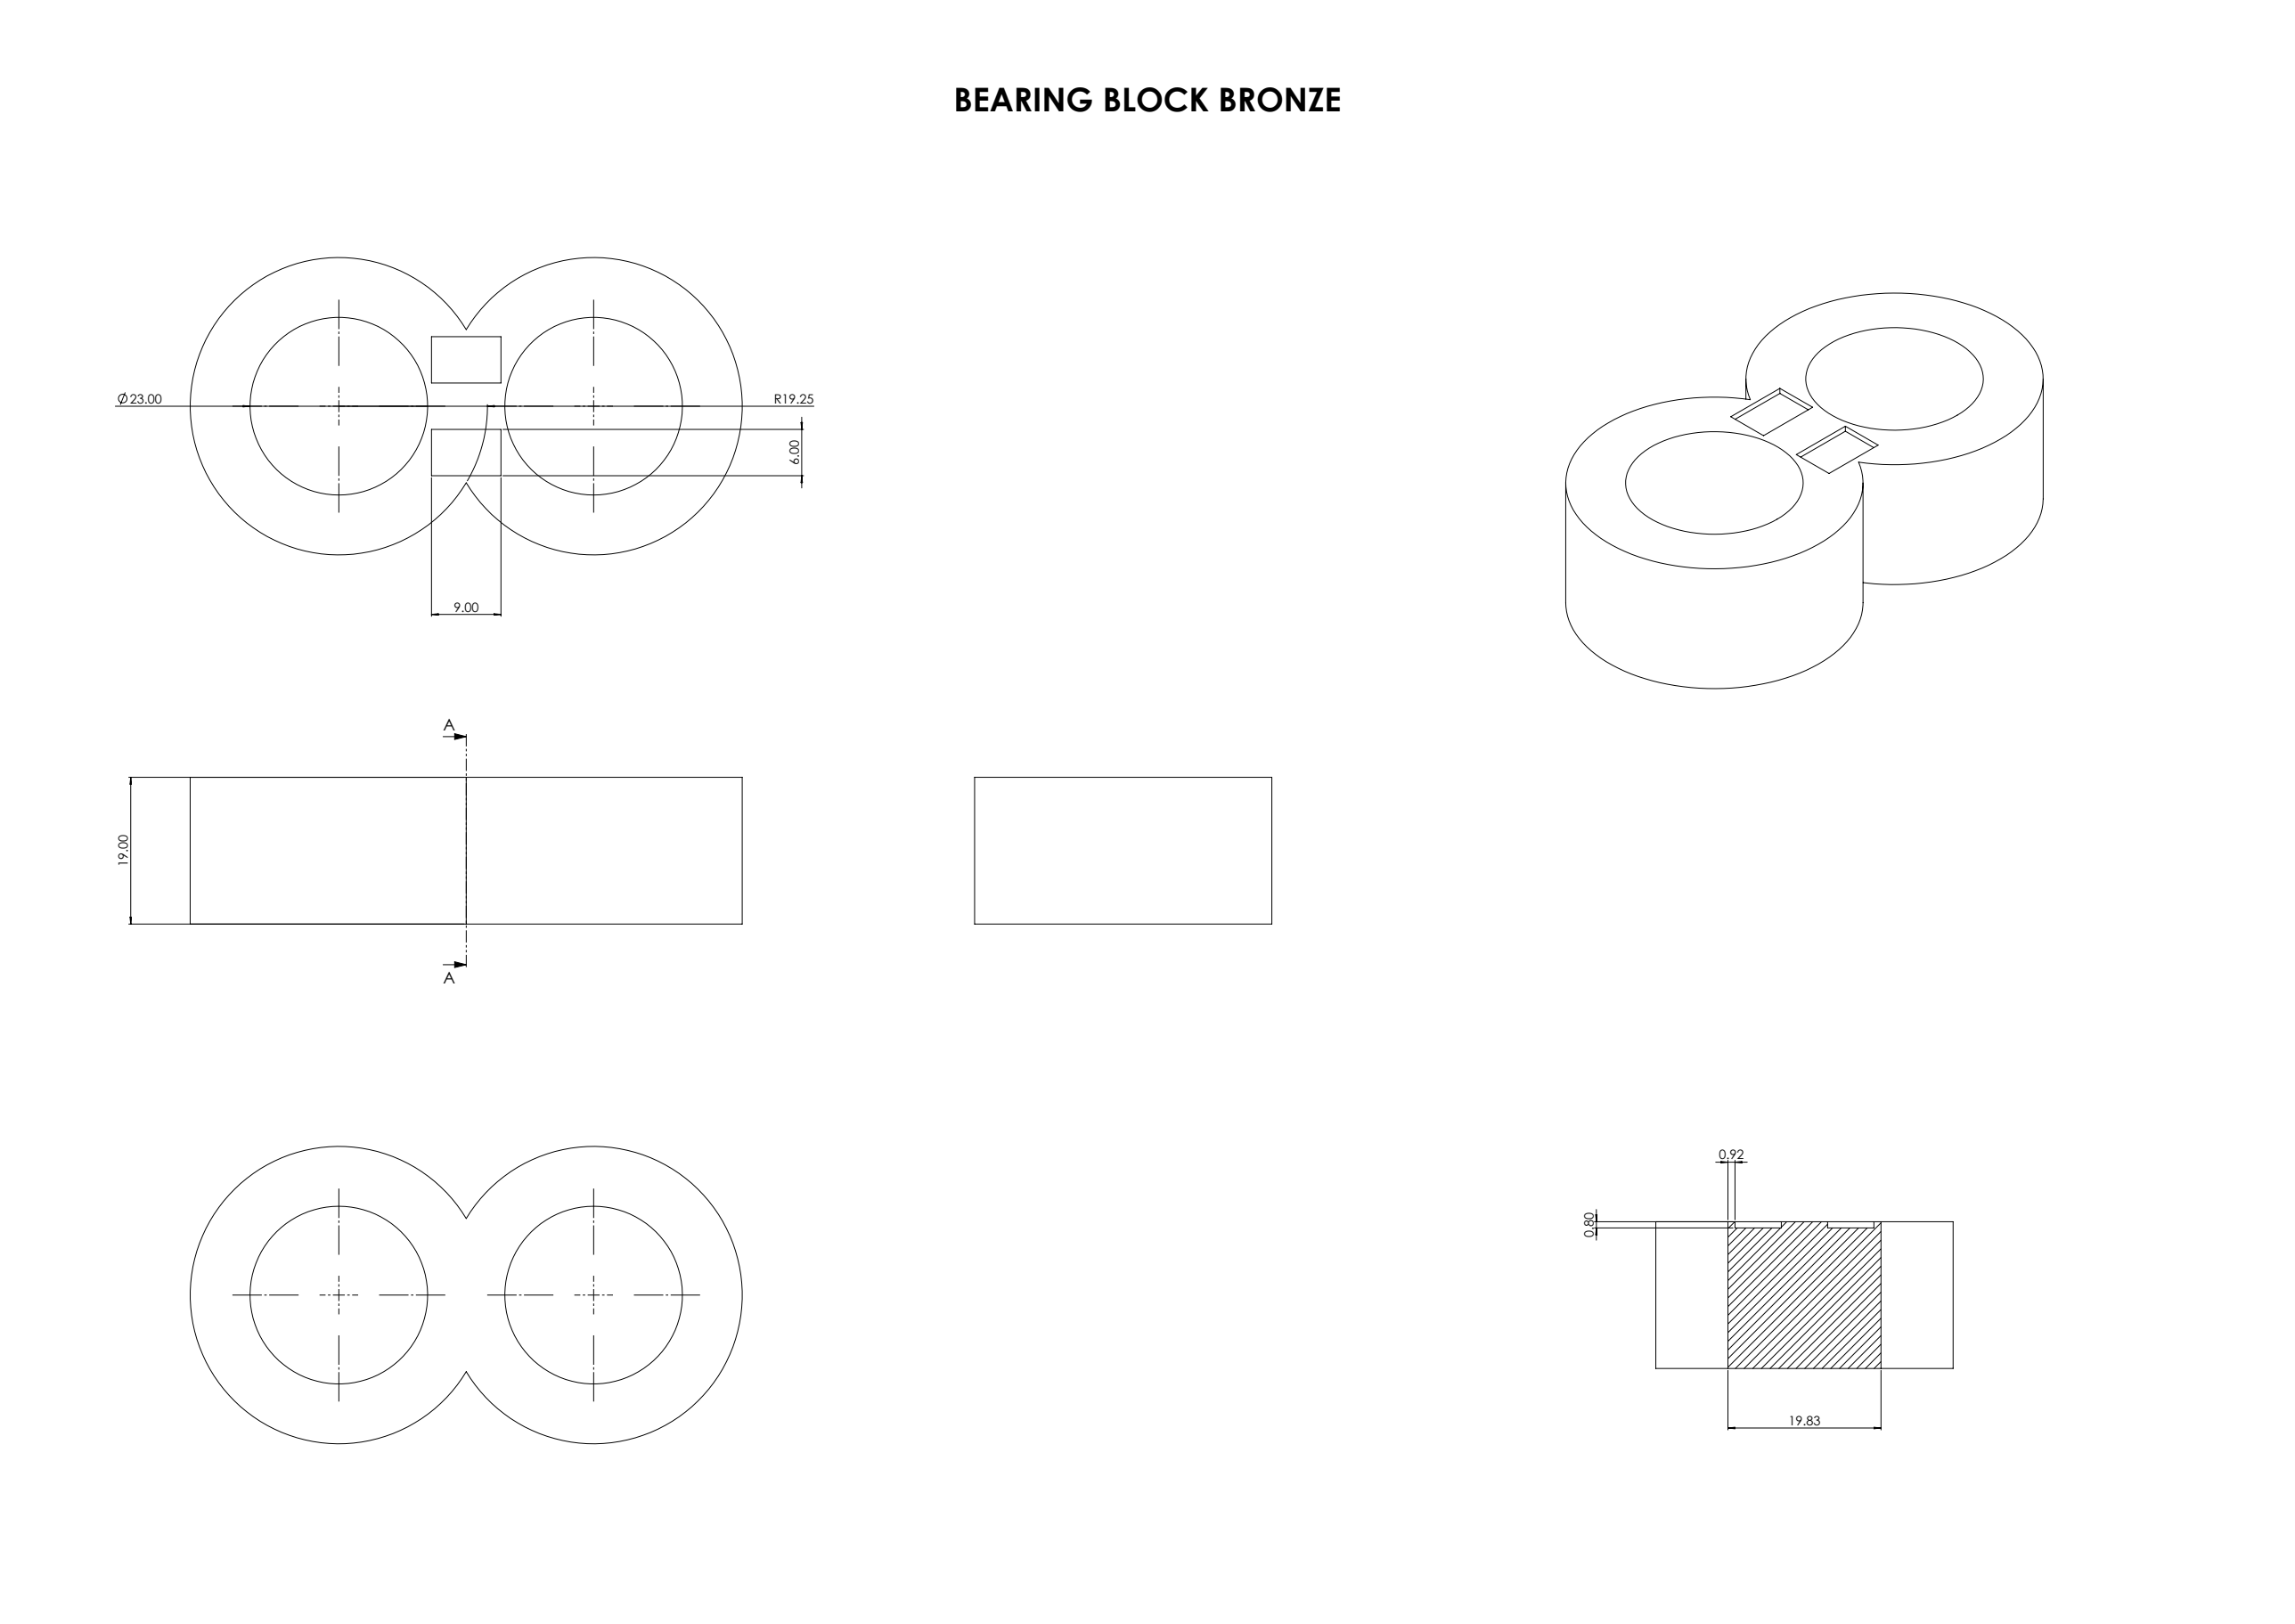
ISO-10303-21;
HEADER;
/* Generated by software containing ST-Developer
 * from STEP Tools, Inc. (www.steptools.com) 
 */

FILE_DESCRIPTION(
/* description */ (''),
/* implementation_level */ '2;1');

FILE_NAME(
/* name */ '06_Bearing_Block_Bronze.step',
/* time_stamp */ '2026-10-26T06:59:52-07:00',
/* author */ (''),
/* organization */ (''),
/* preprocessor_version */ 'ST-DEVELOPER v20.2',
/* originating_system */ 'Autodesk Translation Framework v15.15.0.0',
/* authorisation */ '');

FILE_SCHEMA (('AUTOMOTIVE_DESIGN { 1 0 10303 214 3 1 1 }'));
ENDSEC;

DATA;
#10=MECHANICAL_DESIGN_GEOMETRIC_PRESENTATION_REPRESENTATION('',(#169),#46395);
#141=SHAPE_REPRESENTATION_RELATIONSHIP('SRR','None',#46461,#155);
#155=ADVANCED_BREP_SHAPE_REPRESENTATION('',(#183),#46386);
#169=STYLED_ITEM('',(#46596),#183);
#183=MANIFOLD_SOLID_BREP('Body1',#24942);
#519=CYLINDRICAL_SURFACE('',#26421,11.5);
#520=CYLINDRICAL_SURFACE('',#26424,11.5);
#521=CYLINDRICAL_SURFACE('',#26427,19.25);
#522=CYLINDRICAL_SURFACE('',#26430,19.25);
#651=FACE_BOUND('',#4155,.T.);
#652=FACE_BOUND('',#4156,.T.);
#653=FACE_BOUND('',#4157,.T.);
#654=FACE_BOUND('',#4158,.T.);
#655=FACE_BOUND('',#4160,.T.);
#656=FACE_BOUND('',#4161,.T.);
#1500=PLANE('',#26411);
#1501=PLANE('',#26412);
#1502=PLANE('',#26413);
#1503=PLANE('',#26414);
#1504=PLANE('',#26415);
#1505=PLANE('',#26416);
#1506=PLANE('',#26417);
#1507=PLANE('',#26418);
#1508=PLANE('',#26419);
#1509=PLANE('',#26420);
#1510=PLANE('',#26433);
#1511=PLANE('',#26434);
#2744=FACE_OUTER_BOUND('',#4140,.T.);
#2745=FACE_OUTER_BOUND('',#4141,.T.);
#2746=FACE_OUTER_BOUND('',#4142,.T.);
#2747=FACE_OUTER_BOUND('',#4143,.T.);
#2748=FACE_OUTER_BOUND('',#4144,.T.);
#2749=FACE_OUTER_BOUND('',#4145,.T.);
#2750=FACE_OUTER_BOUND('',#4146,.T.);
#2751=FACE_OUTER_BOUND('',#4147,.T.);
#2752=FACE_OUTER_BOUND('',#4148,.T.);
#2753=FACE_OUTER_BOUND('',#4149,.T.);
#2754=FACE_OUTER_BOUND('',#4150,.T.);
#2755=FACE_OUTER_BOUND('',#4151,.T.);
#2756=FACE_OUTER_BOUND('',#4152,.T.);
#2757=FACE_OUTER_BOUND('',#4153,.T.);
#2758=FACE_OUTER_BOUND('',#4154,.T.);
#2759=FACE_OUTER_BOUND('',#4159,.T.);
#4140=EDGE_LOOP('',(#22016,#22017,#22018,#22019));
#4141=EDGE_LOOP('',(#22020,#22021,#22022,#22023));
#4142=EDGE_LOOP('',(#22024,#22025,#22026,#22027));
#4143=EDGE_LOOP('',(#22028,#22029,#22030,#22031));
#4144=EDGE_LOOP('',(#22032,#22033,#22034,#22035));
#4145=EDGE_LOOP('',(#22036,#22037,#22038,#22039));
#4146=EDGE_LOOP('',(#22040,#22041,#22042,#22043));
#4147=EDGE_LOOP('',(#22044,#22045,#22046,#22047));
#4148=EDGE_LOOP('',(#22048,#22049,#22050,#22051));
#4149=EDGE_LOOP('',(#22052,#22053,#22054,#22055));
#4150=EDGE_LOOP('',(#22056,#22057,#22058,#22059));
#4151=EDGE_LOOP('',(#22060,#22061,#22062,#22063));
#4152=EDGE_LOOP('',(#22064,#22065,#22066,#22067));
#4153=EDGE_LOOP('',(#22068,#22069,#22070,#22071));
#4154=EDGE_LOOP('',(#22072,#22073));
#4155=EDGE_LOOP('',(#22074,#22075,#22076,#22077));
#4156=EDGE_LOOP('',(#22078,#22079,#22080,#22081));
#4157=EDGE_LOOP('',(#22082));
#4158=EDGE_LOOP('',(#22083));
#4159=EDGE_LOOP('',(#22084,#22085));
#4160=EDGE_LOOP('',(#22086));
#4161=EDGE_LOOP('',(#22087));
#6899=LINE('',#40133,#9768);
#6900=LINE('',#40135,#9769);
#6901=LINE('',#40137,#9770);
#6902=LINE('',#40138,#9771);
#6903=LINE('',#40141,#9772);
#6904=LINE('',#40143,#9773);
#6905=LINE('',#40144,#9774);
#6906=LINE('',#40147,#9775);
#6907=LINE('',#40149,#9776);
#6908=LINE('',#40150,#9777);
#6909=LINE('',#40152,#9778);
#6910=LINE('',#40153,#9779);
#6911=LINE('',#40158,#9780);
#6912=LINE('',#40160,#9781);
#6913=LINE('',#40162,#9782);
#6914=LINE('',#40163,#9783);
#6915=LINE('',#40166,#9784);
#6916=LINE('',#40168,#9785);
#6917=LINE('',#40169,#9786);
#6918=LINE('',#40172,#9787);
#6919=LINE('',#40174,#9788);
#6920=LINE('',#40175,#9789);
#6921=LINE('',#40177,#9790);
#6922=LINE('',#40178,#9791);
#6923=LINE('',#40184,#9792);
#6924=LINE('',#40190,#9793);
#6925=LINE('',#40197,#9794);
#6926=LINE('',#40200,#9795);
#9768=VECTOR('',#31910,10.);
#9769=VECTOR('',#31911,10.);
#9770=VECTOR('',#31912,10.);
#9771=VECTOR('',#31913,10.);
#9772=VECTOR('',#31916,10.);
#9773=VECTOR('',#31917,10.);
#9774=VECTOR('',#31918,10.);
#9775=VECTOR('',#31921,10.);
#9776=VECTOR('',#31922,10.);
#9777=VECTOR('',#31923,10.);
#9778=VECTOR('',#31926,10.);
#9779=VECTOR('',#31927,10.);
#9780=VECTOR('',#31932,10.);
#9781=VECTOR('',#31933,10.);
#9782=VECTOR('',#31934,10.);
#9783=VECTOR('',#31935,10.);
#9784=VECTOR('',#31938,10.);
#9785=VECTOR('',#31939,10.);
#9786=VECTOR('',#31940,10.);
#9787=VECTOR('',#31943,10.);
#9788=VECTOR('',#31944,10.);
#9789=VECTOR('',#31945,10.);
#9790=VECTOR('',#31948,10.);
#9791=VECTOR('',#31949,10.);
#9792=VECTOR('',#31956,11.5);
#9793=VECTOR('',#31963,11.5);
#9794=VECTOR('',#31970,10.);
#9795=VECTOR('',#31973,10.);
#10581=CIRCLE('',#26422,11.5);
#10582=CIRCLE('',#26423,11.5);
#10583=CIRCLE('',#26425,11.5);
#10584=CIRCLE('',#26426,11.5);
#10585=CIRCLE('',#26428,19.25);
#10586=CIRCLE('',#26429,19.25);
#10587=CIRCLE('',#26431,19.25);
#10588=CIRCLE('',#26432,19.25);
#12520=VERTEX_POINT('',#40131);
#12521=VERTEX_POINT('',#40132);
#12522=VERTEX_POINT('',#40134);
#12523=VERTEX_POINT('',#40136);
#12524=VERTEX_POINT('',#40140);
#12525=VERTEX_POINT('',#40142);
#12526=VERTEX_POINT('',#40146);
#12527=VERTEX_POINT('',#40148);
#12528=VERTEX_POINT('',#40156);
#12529=VERTEX_POINT('',#40157);
#12530=VERTEX_POINT('',#40159);
#12531=VERTEX_POINT('',#40161);
#12532=VERTEX_POINT('',#40165);
#12533=VERTEX_POINT('',#40167);
#12534=VERTEX_POINT('',#40171);
#12535=VERTEX_POINT('',#40173);
#12536=VERTEX_POINT('',#40181);
#12537=VERTEX_POINT('',#40183);
#12538=VERTEX_POINT('',#40187);
#12539=VERTEX_POINT('',#40189);
#12540=VERTEX_POINT('',#40193);
#12541=VERTEX_POINT('',#40194);
#12542=VERTEX_POINT('',#40196);
#12543=VERTEX_POINT('',#40198);
#15761=EDGE_CURVE('',#12520,#12521,#6899,.T.);
#15762=EDGE_CURVE('',#12520,#12522,#6900,.T.);
#15763=EDGE_CURVE('',#12522,#12523,#6901,.T.);
#15764=EDGE_CURVE('',#12521,#12523,#6902,.T.);
#15765=EDGE_CURVE('',#12524,#12520,#6903,.T.);
#15766=EDGE_CURVE('',#12524,#12525,#6904,.T.);
#15767=EDGE_CURVE('',#12525,#12522,#6905,.T.);
#15768=EDGE_CURVE('',#12526,#12524,#6906,.T.);
#15769=EDGE_CURVE('',#12526,#12527,#6907,.T.);
#15770=EDGE_CURVE('',#12527,#12525,#6908,.T.);
#15771=EDGE_CURVE('',#12521,#12526,#6909,.T.);
#15772=EDGE_CURVE('',#12523,#12527,#6910,.T.);
#15773=EDGE_CURVE('',#12528,#12529,#6911,.T.);
#15774=EDGE_CURVE('',#12528,#12530,#6912,.T.);
#15775=EDGE_CURVE('',#12530,#12531,#6913,.T.);
#15776=EDGE_CURVE('',#12529,#12531,#6914,.T.);
#15777=EDGE_CURVE('',#12532,#12528,#6915,.T.);
#15778=EDGE_CURVE('',#12532,#12533,#6916,.T.);
#15779=EDGE_CURVE('',#12533,#12530,#6917,.T.);
#15780=EDGE_CURVE('',#12534,#12532,#6918,.T.);
#15781=EDGE_CURVE('',#12534,#12535,#6919,.T.);
#15782=EDGE_CURVE('',#12535,#12533,#6920,.T.);
#15783=EDGE_CURVE('',#12529,#12534,#6921,.T.);
#15784=EDGE_CURVE('',#12531,#12535,#6922,.T.);
#15785=EDGE_CURVE('',#12536,#12536,#10581,.T.);
#15786=EDGE_CURVE('',#12536,#12537,#6923,.T.);
#15787=EDGE_CURVE('',#12537,#12537,#10582,.T.);
#15788=EDGE_CURVE('',#12538,#12538,#10583,.T.);
#15789=EDGE_CURVE('',#12538,#12539,#6924,.T.);
#15790=EDGE_CURVE('',#12539,#12539,#10584,.T.);
#15791=EDGE_CURVE('',#12540,#12541,#10585,.T.);
#15792=EDGE_CURVE('',#12541,#12542,#6925,.T.);
#15793=EDGE_CURVE('',#12543,#12542,#10586,.T.);
#15794=EDGE_CURVE('',#12540,#12543,#6926,.T.);
#15795=EDGE_CURVE('',#12541,#12540,#10587,.T.);
#15796=EDGE_CURVE('',#12542,#12543,#10588,.T.);
#22016=ORIENTED_EDGE('',*,*,#15761,.F.);
#22017=ORIENTED_EDGE('',*,*,#15762,.T.);
#22018=ORIENTED_EDGE('',*,*,#15763,.T.);
#22019=ORIENTED_EDGE('',*,*,#15764,.F.);
#22020=ORIENTED_EDGE('',*,*,#15765,.F.);
#22021=ORIENTED_EDGE('',*,*,#15766,.T.);
#22022=ORIENTED_EDGE('',*,*,#15767,.T.);
#22023=ORIENTED_EDGE('',*,*,#15762,.F.);
#22024=ORIENTED_EDGE('',*,*,#15768,.F.);
#22025=ORIENTED_EDGE('',*,*,#15769,.T.);
#22026=ORIENTED_EDGE('',*,*,#15770,.T.);
#22027=ORIENTED_EDGE('',*,*,#15766,.F.);
#22028=ORIENTED_EDGE('',*,*,#15771,.F.);
#22029=ORIENTED_EDGE('',*,*,#15764,.T.);
#22030=ORIENTED_EDGE('',*,*,#15772,.T.);
#22031=ORIENTED_EDGE('',*,*,#15769,.F.);
#22032=ORIENTED_EDGE('',*,*,#15772,.F.);
#22033=ORIENTED_EDGE('',*,*,#15763,.F.);
#22034=ORIENTED_EDGE('',*,*,#15767,.F.);
#22035=ORIENTED_EDGE('',*,*,#15770,.F.);
#22036=ORIENTED_EDGE('',*,*,#15773,.F.);
#22037=ORIENTED_EDGE('',*,*,#15774,.T.);
#22038=ORIENTED_EDGE('',*,*,#15775,.T.);
#22039=ORIENTED_EDGE('',*,*,#15776,.F.);
#22040=ORIENTED_EDGE('',*,*,#15777,.F.);
#22041=ORIENTED_EDGE('',*,*,#15778,.T.);
#22042=ORIENTED_EDGE('',*,*,#15779,.T.);
#22043=ORIENTED_EDGE('',*,*,#15774,.F.);
#22044=ORIENTED_EDGE('',*,*,#15780,.F.);
#22045=ORIENTED_EDGE('',*,*,#15781,.T.);
#22046=ORIENTED_EDGE('',*,*,#15782,.T.);
#22047=ORIENTED_EDGE('',*,*,#15778,.F.);
#22048=ORIENTED_EDGE('',*,*,#15783,.F.);
#22049=ORIENTED_EDGE('',*,*,#15776,.T.);
#22050=ORIENTED_EDGE('',*,*,#15784,.T.);
#22051=ORIENTED_EDGE('',*,*,#15781,.F.);
#22052=ORIENTED_EDGE('',*,*,#15784,.F.);
#22053=ORIENTED_EDGE('',*,*,#15775,.F.);
#22054=ORIENTED_EDGE('',*,*,#15779,.F.);
#22055=ORIENTED_EDGE('',*,*,#15782,.F.);
#22056=ORIENTED_EDGE('',*,*,#15785,.F.);
#22057=ORIENTED_EDGE('',*,*,#15786,.T.);
#22058=ORIENTED_EDGE('',*,*,#15787,.F.);
#22059=ORIENTED_EDGE('',*,*,#15786,.F.);
#22060=ORIENTED_EDGE('',*,*,#15788,.F.);
#22061=ORIENTED_EDGE('',*,*,#15789,.T.);
#22062=ORIENTED_EDGE('',*,*,#15790,.F.);
#22063=ORIENTED_EDGE('',*,*,#15789,.F.);
#22064=ORIENTED_EDGE('',*,*,#15791,.T.);
#22065=ORIENTED_EDGE('',*,*,#15792,.T.);
#22066=ORIENTED_EDGE('',*,*,#15793,.F.);
#22067=ORIENTED_EDGE('',*,*,#15794,.F.);
#22068=ORIENTED_EDGE('',*,*,#15795,.T.);
#22069=ORIENTED_EDGE('',*,*,#15794,.T.);
#22070=ORIENTED_EDGE('',*,*,#15796,.F.);
#22071=ORIENTED_EDGE('',*,*,#15792,.F.);
#22072=ORIENTED_EDGE('',*,*,#15796,.T.);
#22073=ORIENTED_EDGE('',*,*,#15793,.T.);
#22074=ORIENTED_EDGE('',*,*,#15761,.T.);
#22075=ORIENTED_EDGE('',*,*,#15771,.T.);
#22076=ORIENTED_EDGE('',*,*,#15768,.T.);
#22077=ORIENTED_EDGE('',*,*,#15765,.T.);
#22078=ORIENTED_EDGE('',*,*,#15773,.T.);
#22079=ORIENTED_EDGE('',*,*,#15783,.T.);
#22080=ORIENTED_EDGE('',*,*,#15780,.T.);
#22081=ORIENTED_EDGE('',*,*,#15777,.T.);
#22082=ORIENTED_EDGE('',*,*,#15787,.T.);
#22083=ORIENTED_EDGE('',*,*,#15790,.T.);
#22084=ORIENTED_EDGE('',*,*,#15795,.F.);
#22085=ORIENTED_EDGE('',*,*,#15791,.F.);
#22086=ORIENTED_EDGE('',*,*,#15785,.T.);
#22087=ORIENTED_EDGE('',*,*,#15788,.T.);
#24603=ADVANCED_FACE('',(#2744),#1500,.F.);
#24604=ADVANCED_FACE('',(#2745),#1501,.F.);
#24605=ADVANCED_FACE('',(#2746),#1502,.F.);
#24606=ADVANCED_FACE('',(#2747),#1503,.F.);
#24607=ADVANCED_FACE('',(#2748),#1504,.F.);
#24608=ADVANCED_FACE('',(#2749),#1505,.F.);
#24609=ADVANCED_FACE('',(#2750),#1506,.F.);
#24610=ADVANCED_FACE('',(#2751),#1507,.F.);
#24611=ADVANCED_FACE('',(#2752),#1508,.F.);
#24612=ADVANCED_FACE('',(#2753),#1509,.F.);
#24613=ADVANCED_FACE('',(#2754),#519,.F.);
#24614=ADVANCED_FACE('',(#2755),#520,.F.);
#24615=ADVANCED_FACE('',(#2756),#521,.T.);
#24616=ADVANCED_FACE('',(#2757),#522,.T.);
#24617=ADVANCED_FACE('',(#2758,#651,#652,#653,#654),#1510,.T.);
#24618=ADVANCED_FACE('',(#2759,#655,#656),#1511,.F.);
#24942=CLOSED_SHELL('',(#24603,#24604,#24605,#24606,#24607,#24608,#24609,
#24610,#24611,#24612,#24613,#24614,#24615,#24616,#24617,#24618));
#26410=AXIS2_PLACEMENT_3D('',#40129,#31906,#31907);
#26411=AXIS2_PLACEMENT_3D('',#40130,#31908,#31909);
#26412=AXIS2_PLACEMENT_3D('',#40139,#31914,#31915);
#26413=AXIS2_PLACEMENT_3D('',#40145,#31919,#31920);
#26414=AXIS2_PLACEMENT_3D('',#40151,#31924,#31925);
#26415=AXIS2_PLACEMENT_3D('',#40154,#31928,#31929);
#26416=AXIS2_PLACEMENT_3D('',#40155,#31930,#31931);
#26417=AXIS2_PLACEMENT_3D('',#40164,#31936,#31937);
#26418=AXIS2_PLACEMENT_3D('',#40170,#31941,#31942);
#26419=AXIS2_PLACEMENT_3D('',#40176,#31946,#31947);
#26420=AXIS2_PLACEMENT_3D('',#40179,#31950,#31951);
#26421=AXIS2_PLACEMENT_3D('',#40180,#31952,#31953);
#26422=AXIS2_PLACEMENT_3D('',#40182,#31954,#31955);
#26423=AXIS2_PLACEMENT_3D('',#40185,#31957,#31958);
#26424=AXIS2_PLACEMENT_3D('',#40186,#31959,#31960);
#26425=AXIS2_PLACEMENT_3D('',#40188,#31961,#31962);
#26426=AXIS2_PLACEMENT_3D('',#40191,#31964,#31965);
#26427=AXIS2_PLACEMENT_3D('',#40192,#31966,#31967);
#26428=AXIS2_PLACEMENT_3D('',#40195,#31968,#31969);
#26429=AXIS2_PLACEMENT_3D('',#40199,#31971,#31972);
#26430=AXIS2_PLACEMENT_3D('',#40201,#31974,#31975);
#26431=AXIS2_PLACEMENT_3D('',#40202,#31976,#31977);
#26432=AXIS2_PLACEMENT_3D('',#40203,#31978,#31979);
#26433=AXIS2_PLACEMENT_3D('',#40204,#31980,#31981);
#26434=AXIS2_PLACEMENT_3D('',#40205,#31982,#31983);
#31906=DIRECTION('axis',(0.,0.,1.));
#31907=DIRECTION('refdir',(1.,0.,0.));
#31908=DIRECTION('center_axis',(0.,0.,1.));
#31909=DIRECTION('ref_axis',(-1.,0.,0.));
#31910=DIRECTION('',(-1.,0.,0.));
#31911=DIRECTION('',(0.,-1.,0.));
#31912=DIRECTION('',(-1.,0.,0.));
#31913=DIRECTION('',(0.,-1.,0.));
#31914=DIRECTION('center_axis',(1.,0.,0.));
#31915=DIRECTION('ref_axis',(0.,0.,1.));
#31916=DIRECTION('',(0.,0.,1.));
#31917=DIRECTION('',(0.,-1.,0.));
#31918=DIRECTION('',(0.,0.,1.));
#31919=DIRECTION('center_axis',(0.,0.,-1.));
#31920=DIRECTION('ref_axis',(1.,0.,0.));
#31921=DIRECTION('',(1.,0.,0.));
#31922=DIRECTION('',(0.,-1.,0.));
#31923=DIRECTION('',(1.,0.,0.));
#31924=DIRECTION('center_axis',(-1.,0.,0.));
#31925=DIRECTION('ref_axis',(0.,0.,-1.));
#31926=DIRECTION('',(0.,0.,-1.));
#31927=DIRECTION('',(0.,0.,-1.));
#31928=DIRECTION('center_axis',(0.,-1.,0.));
#31929=DIRECTION('ref_axis',(0.,0.,-1.));
#31930=DIRECTION('center_axis',(-1.,0.,0.));
#31931=DIRECTION('ref_axis',(0.,0.,-1.));
#31932=DIRECTION('',(0.,0.,-1.));
#31933=DIRECTION('',(0.,-1.,0.));
#31934=DIRECTION('',(0.,0.,-1.));
#31935=DIRECTION('',(0.,-1.,0.));
#31936=DIRECTION('center_axis',(0.,0.,1.));
#31937=DIRECTION('ref_axis',(-1.,0.,0.));
#31938=DIRECTION('',(-1.,0.,0.));
#31939=DIRECTION('',(0.,-1.,0.));
#31940=DIRECTION('',(-1.,0.,0.));
#31941=DIRECTION('center_axis',(1.,0.,0.));
#31942=DIRECTION('ref_axis',(0.,0.,1.));
#31943=DIRECTION('',(0.,0.,1.));
#31944=DIRECTION('',(0.,-1.,0.));
#31945=DIRECTION('',(0.,0.,1.));
#31946=DIRECTION('center_axis',(0.,0.,-1.));
#31947=DIRECTION('ref_axis',(1.,0.,0.));
#31948=DIRECTION('',(1.,0.,0.));
#31949=DIRECTION('',(1.,0.,0.));
#31950=DIRECTION('center_axis',(0.,-1.,0.));
#31951=DIRECTION('ref_axis',(0.,0.,-1.));
#31952=DIRECTION('center_axis',(0.,1.,0.));
#31953=DIRECTION('ref_axis',(1.,0.,0.));
#31954=DIRECTION('center_axis',(0.,1.,0.));
#31955=DIRECTION('ref_axis',(1.,0.,0.));
#31956=DIRECTION('',(0.,1.,0.));
#31957=DIRECTION('center_axis',(0.,-1.,0.));
#31958=DIRECTION('ref_axis',(1.,0.,0.));
#31959=DIRECTION('center_axis',(0.,1.,0.));
#31960=DIRECTION('ref_axis',(1.,0.,0.));
#31961=DIRECTION('center_axis',(0.,1.,0.));
#31962=DIRECTION('ref_axis',(1.,0.,0.));
#31963=DIRECTION('',(0.,1.,0.));
#31964=DIRECTION('center_axis',(0.,-1.,0.));
#31965=DIRECTION('ref_axis',(1.,0.,0.));
#31966=DIRECTION('center_axis',(0.,1.,0.));
#31967=DIRECTION('ref_axis',(-1.83697019872103E-16,0.,1.));
#31968=DIRECTION('center_axis',(0.,1.,0.));
#31969=DIRECTION('ref_axis',(1.,0.,0.));
#31970=DIRECTION('',(0.,1.,0.));
#31971=DIRECTION('center_axis',(0.,1.,0.));
#31972=DIRECTION('ref_axis',(1.,0.,0.));
#31973=DIRECTION('',(0.,1.,0.));
#31974=DIRECTION('center_axis',(0.,1.,0.));
#31975=DIRECTION('ref_axis',(-1.60812264967664E-16,0.,-1.));
#31976=DIRECTION('center_axis',(0.,1.,0.));
#31977=DIRECTION('ref_axis',(1.,0.,0.));
#31978=DIRECTION('center_axis',(0.,1.,0.));
#31979=DIRECTION('ref_axis',(1.,0.,0.));
#31980=DIRECTION('center_axis',(0.,1.,0.));
#31981=DIRECTION('ref_axis',(1.,0.,0.));
#31982=DIRECTION('center_axis',(0.,1.,0.));
#31983=DIRECTION('ref_axis',(1.,0.,0.));
#40129=CARTESIAN_POINT('',(0.,0.,0.));
#40130=CARTESIAN_POINT('Origin',(9.,37.,-12.));
#40131=CARTESIAN_POINT('',(9.,37.,-12.));
#40132=CARTESIAN_POINT('',(3.,37.,-12.));
#40133=CARTESIAN_POINT('',(4.5,37.,-12.));
#40134=CARTESIAN_POINT('',(9.,36.2,-12.));
#40135=CARTESIAN_POINT('',(9.,37.,-12.));
#40136=CARTESIAN_POINT('',(3.,36.2,-12.));
#40137=CARTESIAN_POINT('',(3.,36.2,-12.));
#40138=CARTESIAN_POINT('',(3.,37.,-12.));
#40139=CARTESIAN_POINT('Origin',(9.,37.,-21.));
#40140=CARTESIAN_POINT('',(9.,37.,-21.));
#40141=CARTESIAN_POINT('',(9.,37.,-18.75));
#40142=CARTESIAN_POINT('',(9.,36.2,-21.));
#40143=CARTESIAN_POINT('',(9.,37.,-21.));
#40144=CARTESIAN_POINT('',(9.,36.2,-12.));
#40145=CARTESIAN_POINT('Origin',(3.,37.,-21.));
#40146=CARTESIAN_POINT('',(3.,37.,-21.));
#40147=CARTESIAN_POINT('',(1.5,37.,-21.));
#40148=CARTESIAN_POINT('',(3.,36.2,-21.));
#40149=CARTESIAN_POINT('',(3.,37.,-21.));
#40150=CARTESIAN_POINT('',(9.,36.2,-21.));
#40151=CARTESIAN_POINT('Origin',(3.,37.,-12.));
#40152=CARTESIAN_POINT('',(3.,37.,-14.25));
#40153=CARTESIAN_POINT('',(3.,36.2,-21.));
#40154=CARTESIAN_POINT('Origin',(6.,36.2,-16.5));
#40155=CARTESIAN_POINT('Origin',(-9.,37.,-12.));
#40156=CARTESIAN_POINT('',(-9.,37.,-12.));
#40157=CARTESIAN_POINT('',(-9.,37.,-21.));
#40158=CARTESIAN_POINT('',(-9.,37.,-14.25));
#40159=CARTESIAN_POINT('',(-9.,36.2,-12.));
#40160=CARTESIAN_POINT('',(-9.,37.,-12.));
#40161=CARTESIAN_POINT('',(-9.,36.2,-21.));
#40162=CARTESIAN_POINT('',(-9.,36.2,-12.));
#40163=CARTESIAN_POINT('',(-9.,37.,-21.));
#40164=CARTESIAN_POINT('Origin',(-3.,37.,-12.));
#40165=CARTESIAN_POINT('',(-3.,37.,-12.));
#40166=CARTESIAN_POINT('',(-1.5,37.,-12.));
#40167=CARTESIAN_POINT('',(-3.,36.2,-12.));
#40168=CARTESIAN_POINT('',(-3.,37.,-12.));
#40169=CARTESIAN_POINT('',(-3.,36.2,-12.));
#40170=CARTESIAN_POINT('Origin',(-3.,37.,-21.));
#40171=CARTESIAN_POINT('',(-3.,37.,-21.));
#40172=CARTESIAN_POINT('',(-3.,37.,-18.75));
#40173=CARTESIAN_POINT('',(-3.,36.2,-21.));
#40174=CARTESIAN_POINT('',(-3.,37.,-21.));
#40175=CARTESIAN_POINT('',(-3.,36.2,-21.));
#40176=CARTESIAN_POINT('Origin',(-9.,37.,-21.));
#40177=CARTESIAN_POINT('',(-4.5,37.,-21.));
#40178=CARTESIAN_POINT('',(-9.,36.2,-21.));
#40179=CARTESIAN_POINT('Origin',(-6.,36.2,-16.5));
#40180=CARTESIAN_POINT('Origin',(0.,18.,0.));
#40181=CARTESIAN_POINT('',(-11.5,18.,1.40834381901946E-15));
#40182=CARTESIAN_POINT('Origin',(0.,18.,0.));
#40183=CARTESIAN_POINT('',(-11.5,37.,1.40834381901946E-15));
#40184=CARTESIAN_POINT('',(-11.5,18.,1.40834381901946E-15));
#40185=CARTESIAN_POINT('Origin',(0.,37.,0.));
#40186=CARTESIAN_POINT('Origin',(0.,18.,-33.));
#40187=CARTESIAN_POINT('',(-11.5,18.,-33.));
#40188=CARTESIAN_POINT('Origin',(0.,18.,-33.));
#40189=CARTESIAN_POINT('',(-11.5,37.,-33.));
#40190=CARTESIAN_POINT('',(-11.5,18.,-33.));
#40191=CARTESIAN_POINT('Origin',(0.,37.,-33.));
#40192=CARTESIAN_POINT('Origin',(0.,18.,0.));
#40193=CARTESIAN_POINT('',(-9.91526600752597,18.,-16.5));
#40194=CARTESIAN_POINT('',(9.91526600752597,18.,-16.5));
#40195=CARTESIAN_POINT('Origin',(0.,18.,0.));
#40196=CARTESIAN_POINT('',(9.91526600752597,37.,-16.5));
#40197=CARTESIAN_POINT('',(9.91526600752597,18.,-16.5));
#40198=CARTESIAN_POINT('',(-9.91526600752597,37.,-16.5));
#40199=CARTESIAN_POINT('Origin',(0.,37.,0.));
#40200=CARTESIAN_POINT('',(-9.91526600752597,18.,-16.5));
#40201=CARTESIAN_POINT('Origin',(0.,18.,-33.));
#40202=CARTESIAN_POINT('Origin',(0.,18.,-33.));
#40203=CARTESIAN_POINT('Origin',(0.,37.,-33.));
#40204=CARTESIAN_POINT('Origin',(0.,37.,-16.5));
#40205=CARTESIAN_POINT('Origin',(0.,18.,-16.5));
#46370=UNCERTAINTY_MEASURE_WITH_UNIT(LENGTH_MEASURE(0.01),#46396,
'DISTANCE_ACCURACY_VALUE',
'Maximum model space distance between geometric entities at asserted c
onnectivities');
#46379=UNCERTAINTY_MEASURE_WITH_UNIT(LENGTH_MEASURE(0.01),#46396,
'DISTANCE_ACCURACY_VALUE',
'Maximum model space distance between geometric entities at asserted c
onnectivities');
#46386=(
GEOMETRIC_REPRESENTATION_CONTEXT(3)
GLOBAL_UNCERTAINTY_ASSIGNED_CONTEXT((#46370))
GLOBAL_UNIT_ASSIGNED_CONTEXT((#46396,#46398,#46399))
REPRESENTATION_CONTEXT('','3D')
);
#46395=(
GEOMETRIC_REPRESENTATION_CONTEXT(3)
GLOBAL_UNCERTAINTY_ASSIGNED_CONTEXT((#46379))
GLOBAL_UNIT_ASSIGNED_CONTEXT((#46396,#46398,#46399))
REPRESENTATION_CONTEXT('','3D')
);
#46396=(
LENGTH_UNIT()
NAMED_UNIT(*)
SI_UNIT(.MILLI.,.METRE.)
);
#46398=(
NAMED_UNIT(*)
PLANE_ANGLE_UNIT()
SI_UNIT($,.RADIAN.)
);
#46399=(
NAMED_UNIT(*)
SI_UNIT($,.STERADIAN.)
SOLID_ANGLE_UNIT()
);
#46406=SHAPE_DEFINITION_REPRESENTATION(#46421,#46461);
#46421=PRODUCT_DEFINITION_SHAPE('',$,#46477);
#46461=SHAPE_REPRESENTATION('',(#26410),#46386);
#46470=PRODUCT_DEFINITION_CONTEXT('part definition',#46517,'design');
#46477=PRODUCT_DEFINITION('2026-10-26-00-51-10-414',
'06_Bearing_Block_Bronze',#46492,#46470);
#46492=PRODUCT_DEFINITION_FORMATION('',$,#46525);
#46517=APPLICATION_CONTEXT(
'Core Data for Automotive Mechanical Design Process');
#46518=PRODUCT_CONTEXT('part definition',#46517,'mechanical');
#46525=PRODUCT('2026-10-26-00-51-10-414','06_Bearing_Block_Bronze',$,(#46518));
#46590=COLOUR_RGB('Grey',0.48,0.52,0.57);
#46591=FILL_AREA_STYLE_COLOUR('',#46590);
#46592=FILL_AREA_STYLE('',(#46591));
#46593=SURFACE_STYLE_FILL_AREA(#46592);
#46594=SURFACE_SIDE_STYLE('',(#46593));
#46595=SURFACE_STYLE_USAGE(.BOTH.,#46594);
#46596=PRESENTATION_STYLE_ASSIGNMENT((#46595));
ENDSEC;
END-ISO-10303-21;
